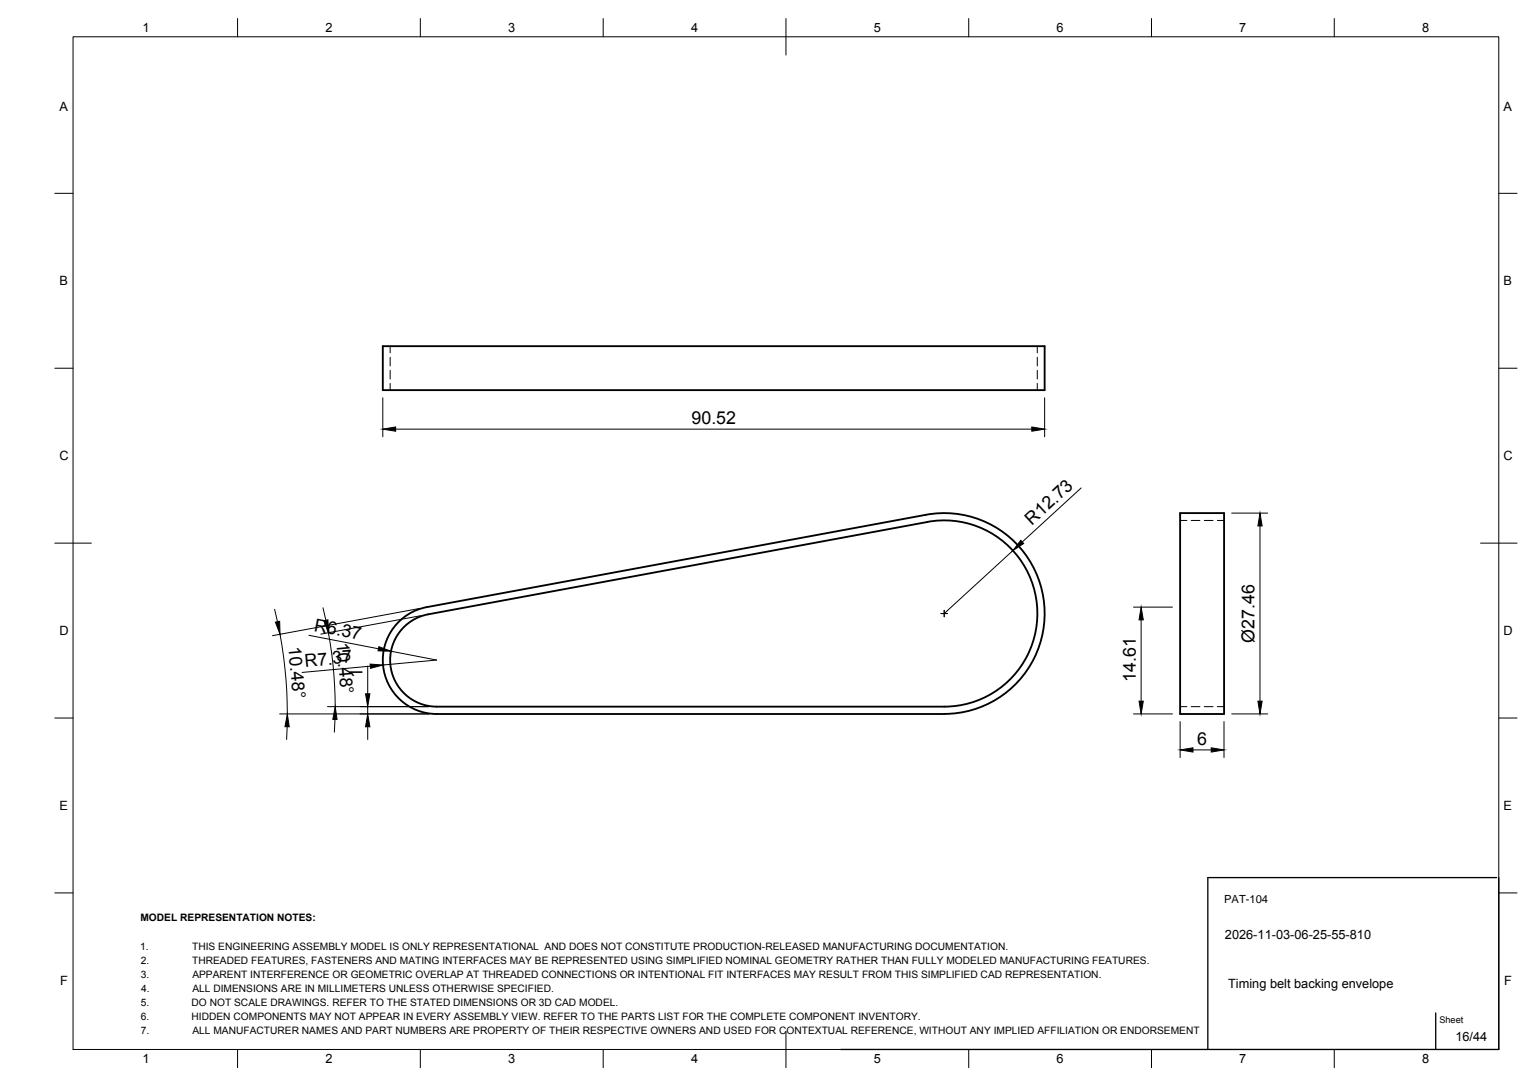
ISO-10303-21;
HEADER;
/* Generated by software containing ST-Developer
 * from STEP Tools, Inc. (www.steptools.com) 
 */

FILE_DESCRIPTION(
/* description */ ('Timing belt drive module 2 mm Pitch Timing 20T-40T'),

/* implementation_level */ '2;1');

FILE_NAME(
/* name */ 'Timing belt backing envelope.step',
/* time_stamp */ '2026-10-28T03:25:12-07:00',
/* author */ (''),
/* organization */ (''),
/* preprocessor_version */ 'ST-DEVELOPER v20.2',
/* originating_system */ 'Autodesk Translation Framework v15.17.0.0',
/* authorisation */ '');

FILE_SCHEMA (('AUTOMOTIVE_DESIGN { 1 0 10303 214 3 1 1 }'));
ENDSEC;

DATA;
#10=MECHANICAL_DESIGN_GEOMETRIC_PRESENTATION_REPRESENTATION('',(#539),#17830);
#453=SHAPE_REPRESENTATION_RELATIONSHIP('SRR','None',#18023,#496);
#496=ADVANCED_BREP_SHAPE_REPRESENTATION('',(#597),#17798);
#539=STYLED_ITEM('',(#18324),#597);
#597=MANIFOLD_SOLID_BREP('Body1',#8996);
#707=FACE_BOUND('',#1712,.T.);
#708=FACE_BOUND('',#1720,.T.);
#847=PLANE('',#9858);
#848=PLANE('',#9859);
#849=PLANE('',#9860);
#850=PLANE('',#9871);
#851=PLANE('',#9872);
#852=PLANE('',#9875);
#1118=FACE_OUTER_BOUND('',#1709,.T.);
#1119=FACE_OUTER_BOUND('',#1710,.T.);
#1120=FACE_OUTER_BOUND('',#1711,.T.);
#1121=FACE_OUTER_BOUND('',#1713,.T.);
#1122=FACE_OUTER_BOUND('',#1714,.T.);
#1123=FACE_OUTER_BOUND('',#1715,.T.);
#1124=FACE_OUTER_BOUND('',#1716,.T.);
#1125=FACE_OUTER_BOUND('',#1717,.T.);
#1126=FACE_OUTER_BOUND('',#1718,.T.);
#1127=FACE_OUTER_BOUND('',#1719,.T.);
#1709=EDGE_LOOP('',(#6493,#6494,#6495,#6496));
#1710=EDGE_LOOP('',(#6497,#6498,#6499,#6500));
#1711=EDGE_LOOP('',(#6501,#6502,#6503,#6504));
#1712=EDGE_LOOP('',(#6505,#6506,#6507,#6508));
#1713=EDGE_LOOP('',(#6509,#6510,#6511,#6512));
#1714=EDGE_LOOP('',(#6513,#6514,#6515,#6516));
#1715=EDGE_LOOP('',(#6517,#6518,#6519,#6520));
#1716=EDGE_LOOP('',(#6521,#6522,#6523,#6524));
#1717=EDGE_LOOP('',(#6525,#6526,#6527,#6528));
#1718=EDGE_LOOP('',(#6529,#6530,#6531,#6532));
#1719=EDGE_LOOP('',(#6533,#6534,#6535,#6536));
#1720=EDGE_LOOP('',(#6537,#6538,#6539,#6540));
#2308=CIRCLE('',#9861,0.736619772367581);
#2309=CIRCLE('',#9862,1.37323954473516);
#2310=CIRCLE('',#9863,0.636619772367581);
#2311=CIRCLE('',#9864,1.27323954473516);
#2312=CIRCLE('',#9866,0.636619772367581);
#2313=CIRCLE('',#9868,1.27323954473516);
#2314=CIRCLE('',#9870,1.37323954473516);
#2315=CIRCLE('',#9874,0.736619772367581);
#2982=LINE('',#14650,#3460);
#2983=LINE('',#14652,#3461);
#2984=LINE('',#14654,#3462);
#2985=LINE('',#14655,#3463);
#2986=LINE('',#14659,#3464);
#2987=LINE('',#14661,#3465);
#2988=LINE('',#14663,#3466);
#2989=LINE('',#14664,#3467);
#2990=LINE('',#14668,#3468);
#2991=LINE('',#14672,#3469);
#2992=LINE('',#14682,#3470);
#2993=LINE('',#14685,#3471);
#2994=LINE('',#14688,#3472);
#2995=LINE('',#14689,#3473);
#2996=LINE('',#14692,#3474);
#2997=LINE('',#14693,#3475);
#3460=VECTOR('',#11687,1.);
#3461=VECTOR('',#11688,1.);
#3462=VECTOR('',#11689,1.);
#3463=VECTOR('',#11690,1.);
#3464=VECTOR('',#11693,1.);
#3465=VECTOR('',#11694,1.);
#3466=VECTOR('',#11695,1.);
#3467=VECTOR('',#11696,1.);
#3468=VECTOR('',#11699,1.);
#3469=VECTOR('',#11702,1.);
#3470=VECTOR('',#11719,1.);
#3471=VECTOR('',#11722,1.);
#3472=VECTOR('',#11725,1.);
#3473=VECTOR('',#11726,1.);
#3474=VECTOR('',#11729,1.);
#3475=VECTOR('',#11730,1.);
#3986=VERTEX_POINT('',#14648);
#3987=VERTEX_POINT('',#14649);
#3988=VERTEX_POINT('',#14651);
#3989=VERTEX_POINT('',#14653);
#3990=VERTEX_POINT('',#14657);
#3991=VERTEX_POINT('',#14658);
#3992=VERTEX_POINT('',#14660);
#3993=VERTEX_POINT('',#14662);
#3994=VERTEX_POINT('',#14666);
#3995=VERTEX_POINT('',#14667);
#3996=VERTEX_POINT('',#14669);
#3997=VERTEX_POINT('',#14671);
#3998=VERTEX_POINT('',#14681);
#3999=VERTEX_POINT('',#14683);
#4000=VERTEX_POINT('',#14687);
#4001=VERTEX_POINT('',#14691);
#4929=EDGE_CURVE('',#3986,#3987,#2982,.T.);
#4930=EDGE_CURVE('',#3988,#3986,#2983,.T.);
#4931=EDGE_CURVE('',#3989,#3988,#2984,.T.);
#4932=EDGE_CURVE('',#3989,#3987,#2985,.T.);
#4933=EDGE_CURVE('',#3990,#3991,#2986,.T.);
#4934=EDGE_CURVE('',#3992,#3990,#2987,.T.);
#4935=EDGE_CURVE('',#3993,#3992,#2988,.T.);
#4936=EDGE_CURVE('',#3991,#3993,#2989,.T.);
#4937=EDGE_CURVE('',#3994,#3995,#2990,.T.);
#4938=EDGE_CURVE('',#3996,#3994,#2308,.T.);
#4939=EDGE_CURVE('',#3997,#3996,#2991,.T.);
#4940=EDGE_CURVE('',#3995,#3997,#2309,.T.);
#4941=EDGE_CURVE('',#3987,#3990,#2310,.T.);
#4942=EDGE_CURVE('',#3991,#3986,#2311,.T.);
#4943=EDGE_CURVE('',#3992,#3989,#2312,.T.);
#4944=EDGE_CURVE('',#3988,#3993,#2313,.T.);
#4945=EDGE_CURVE('',#3997,#3998,#2992,.T.);
#4946=EDGE_CURVE('',#3999,#3998,#2314,.T.);
#4947=EDGE_CURVE('',#3995,#3999,#2993,.T.);
#4948=EDGE_CURVE('',#3996,#4000,#2994,.T.);
#4949=EDGE_CURVE('',#3998,#4000,#2995,.T.);
#4950=EDGE_CURVE('',#4001,#3999,#2996,.T.);
#4951=EDGE_CURVE('',#3994,#4001,#2997,.T.);
#4952=EDGE_CURVE('',#4000,#4001,#2315,.T.);
#6493=ORIENTED_EDGE('',*,*,#4929,.F.);
#6494=ORIENTED_EDGE('',*,*,#4930,.F.);
#6495=ORIENTED_EDGE('',*,*,#4931,.F.);
#6496=ORIENTED_EDGE('',*,*,#4932,.T.);
#6497=ORIENTED_EDGE('',*,*,#4933,.F.);
#6498=ORIENTED_EDGE('',*,*,#4934,.F.);
#6499=ORIENTED_EDGE('',*,*,#4935,.F.);
#6500=ORIENTED_EDGE('',*,*,#4936,.F.);
#6501=ORIENTED_EDGE('',*,*,#4937,.F.);
#6502=ORIENTED_EDGE('',*,*,#4938,.F.);
#6503=ORIENTED_EDGE('',*,*,#4939,.F.);
#6504=ORIENTED_EDGE('',*,*,#4940,.F.);
#6505=ORIENTED_EDGE('',*,*,#4929,.T.);
#6506=ORIENTED_EDGE('',*,*,#4941,.T.);
#6507=ORIENTED_EDGE('',*,*,#4933,.T.);
#6508=ORIENTED_EDGE('',*,*,#4942,.T.);
#6509=ORIENTED_EDGE('',*,*,#4932,.F.);
#6510=ORIENTED_EDGE('',*,*,#4943,.F.);
#6511=ORIENTED_EDGE('',*,*,#4934,.T.);
#6512=ORIENTED_EDGE('',*,*,#4941,.F.);
#6513=ORIENTED_EDGE('',*,*,#4930,.T.);
#6514=ORIENTED_EDGE('',*,*,#4942,.F.);
#6515=ORIENTED_EDGE('',*,*,#4936,.T.);
#6516=ORIENTED_EDGE('',*,*,#4944,.F.);
#6517=ORIENTED_EDGE('',*,*,#4945,.T.);
#6518=ORIENTED_EDGE('',*,*,#4946,.F.);
#6519=ORIENTED_EDGE('',*,*,#4947,.F.);
#6520=ORIENTED_EDGE('',*,*,#4940,.T.);
#6521=ORIENTED_EDGE('',*,*,#4939,.T.);
#6522=ORIENTED_EDGE('',*,*,#4948,.T.);
#6523=ORIENTED_EDGE('',*,*,#4949,.F.);
#6524=ORIENTED_EDGE('',*,*,#4945,.F.);
#6525=ORIENTED_EDGE('',*,*,#4937,.T.);
#6526=ORIENTED_EDGE('',*,*,#4947,.T.);
#6527=ORIENTED_EDGE('',*,*,#4950,.F.);
#6528=ORIENTED_EDGE('',*,*,#4951,.F.);
#6529=ORIENTED_EDGE('',*,*,#4948,.F.);
#6530=ORIENTED_EDGE('',*,*,#4938,.T.);
#6531=ORIENTED_EDGE('',*,*,#4951,.T.);
#6532=ORIENTED_EDGE('',*,*,#4952,.F.);
#6533=ORIENTED_EDGE('',*,*,#4949,.T.);
#6534=ORIENTED_EDGE('',*,*,#4952,.T.);
#6535=ORIENTED_EDGE('',*,*,#4950,.T.);
#6536=ORIENTED_EDGE('',*,*,#4946,.T.);
#6537=ORIENTED_EDGE('',*,*,#4931,.T.);
#6538=ORIENTED_EDGE('',*,*,#4944,.T.);
#6539=ORIENTED_EDGE('',*,*,#4935,.T.);
#6540=ORIENTED_EDGE('',*,*,#4943,.T.);
#8263=CYLINDRICAL_SURFACE('',#9865,0.636619772367581);
#8264=CYLINDRICAL_SURFACE('',#9867,1.27323954473516);
#8265=CYLINDRICAL_SURFACE('',#9869,1.37323954473516);
#8266=CYLINDRICAL_SURFACE('',#9873,0.736619772367581);
#8616=ADVANCED_FACE('',(#1118),#847,.F.);
#8617=ADVANCED_FACE('',(#1119),#848,.F.);
#8618=ADVANCED_FACE('',(#1120,#707),#849,.F.);
#8619=ADVANCED_FACE('',(#1121),#8263,.F.);
#8620=ADVANCED_FACE('',(#1122),#8264,.F.);
#8621=ADVANCED_FACE('',(#1123),#8265,.T.);
#8622=ADVANCED_FACE('',(#1124),#850,.T.);
#8623=ADVANCED_FACE('',(#1125),#851,.T.);
#8624=ADVANCED_FACE('',(#1126),#8266,.T.);
#8625=ADVANCED_FACE('',(#1127,#708),#852,.T.);
#8996=CLOSED_SHELL('',(#8616,#8617,#8618,#8619,#8620,#8621,#8622,#8623,
#8624,#8625));
#9857=AXIS2_PLACEMENT_3D('',#14646,#11683,#11684);
#9858=AXIS2_PLACEMENT_3D('',#14647,#11685,#11686);
#9859=AXIS2_PLACEMENT_3D('',#14656,#11691,#11692);
#9860=AXIS2_PLACEMENT_3D('',#14665,#11697,#11698);
#9861=AXIS2_PLACEMENT_3D('',#14670,#11700,#11701);
#9862=AXIS2_PLACEMENT_3D('',#14673,#11703,#11704);
#9863=AXIS2_PLACEMENT_3D('',#14674,#11705,#11706);
#9864=AXIS2_PLACEMENT_3D('',#14675,#11707,#11708);
#9865=AXIS2_PLACEMENT_3D('',#14676,#11709,#11710);
#9866=AXIS2_PLACEMENT_3D('',#14677,#11711,#11712);
#9867=AXIS2_PLACEMENT_3D('',#14678,#11713,#11714);
#9868=AXIS2_PLACEMENT_3D('',#14679,#11715,#11716);
#9869=AXIS2_PLACEMENT_3D('',#14680,#11717,#11718);
#9870=AXIS2_PLACEMENT_3D('',#14684,#11720,#11721);
#9871=AXIS2_PLACEMENT_3D('',#14686,#11723,#11724);
#9872=AXIS2_PLACEMENT_3D('',#14690,#11727,#11728);
#9873=AXIS2_PLACEMENT_3D('',#14694,#11731,#11732);
#9874=AXIS2_PLACEMENT_3D('',#14695,#11733,#11734);
#9875=AXIS2_PLACEMENT_3D('',#14696,#11735,#11736);
#11683=DIRECTION('axis',(0.,0.,1.));
#11684=DIRECTION('refdir',(1.,0.,0.));
#11685=DIRECTION('center_axis',(-0.0913252028230577,0.,-0.99582112215464));
#11686=DIRECTION('ref_axis',(-0.99582112215464,0.,0.0913252028230577));
#11687=DIRECTION('',(-0.99582112215464,0.,0.0913252028230577));
#11688=DIRECTION('',(0.,-1.,0.));
#11689=DIRECTION('',(0.99582112215464,0.,-0.0913252028230577));
#11690=DIRECTION('',(0.,-1.,0.));
#11691=DIRECTION('center_axis',(-0.0913252028230577,0.,0.99582112215464));
#11692=DIRECTION('ref_axis',(0.99582112215464,0.,0.0913252028230577));
#11693=DIRECTION('',(0.99582112215464,0.,0.0913252028230577));
#11694=DIRECTION('',(0.,-1.,0.));
#11695=DIRECTION('',(-0.99582112215464,0.,-0.0913252028230577));
#11696=DIRECTION('',(0.,1.,0.));
#11697=DIRECTION('center_axis',(0.,1.,0.));
#11698=DIRECTION('ref_axis',(1.,0.,0.));
#11699=DIRECTION('',(0.99582112215464,0.,0.091325202823058));
#11700=DIRECTION('center_axis',(0.,1.,0.));
#11701=DIRECTION('ref_axis',(1.,0.,0.));
#11702=DIRECTION('',(-0.99582112215464,0.,0.0913252028230577));
#11703=DIRECTION('center_axis',(0.,1.,0.));
#11704=DIRECTION('ref_axis',(1.,0.,0.));
#11705=DIRECTION('center_axis',(0.,1.,0.));
#11706=DIRECTION('ref_axis',(1.,0.,0.));
#11707=DIRECTION('center_axis',(0.,1.,0.));
#11708=DIRECTION('ref_axis',(1.,0.,0.));
#11709=DIRECTION('center_axis',(0.,1.,0.));
#11710=DIRECTION('ref_axis',(-1.,0.,-1.22464679914735E-16));
#11711=DIRECTION('center_axis',(0.,-1.,0.));
#11712=DIRECTION('ref_axis',(1.,0.,0.));
#11713=DIRECTION('center_axis',(0.,1.,0.));
#11714=DIRECTION('ref_axis',(1.,0.,0.));
#11715=DIRECTION('center_axis',(0.,-1.,0.));
#11716=DIRECTION('ref_axis',(1.,0.,0.));
#11717=DIRECTION('center_axis',(0.,1.,0.));
#11718=DIRECTION('ref_axis',(1.,0.,0.));
#11719=DIRECTION('',(0.,1.,0.));
#11720=DIRECTION('center_axis',(0.,1.,0.));
#11721=DIRECTION('ref_axis',(1.,0.,0.));
#11722=DIRECTION('',(0.,1.,0.));
#11723=DIRECTION('center_axis',(-0.0913252028230577,0.,-0.99582112215464));
#11724=DIRECTION('ref_axis',(-0.99582112215464,0.,0.0913252028230577));
#11725=DIRECTION('',(0.,1.,0.));
#11726=DIRECTION('',(-0.99582112215464,0.,0.0913252028230577));
#11727=DIRECTION('center_axis',(-0.091325202823058,0.,0.99582112215464));
#11728=DIRECTION('ref_axis',(0.99582112215464,0.,0.091325202823058));
#11729=DIRECTION('',(0.99582112215464,0.,0.091325202823058));
#11730=DIRECTION('',(0.,1.,0.));
#11731=DIRECTION('center_axis',(0.,1.,0.));
#11732=DIRECTION('ref_axis',(-1.,0.,-1.22464679914735E-16));
#11733=DIRECTION('center_axis',(0.,1.,0.));
#11734=DIRECTION('ref_axis',(1.,0.,0.));
#11735=DIRECTION('center_axis',(0.,1.,0.));
#11736=DIRECTION('ref_axis',(1.,0.,0.));
#14646=CARTESIAN_POINT('',(0.,0.,0.));
#14647=CARTESIAN_POINT('Origin',(6.85463117051588,-3.5,5.73208116779017));
#14648=CARTESIAN_POINT('',(6.85463117051588,-3.425,5.73208116779017));
#14649=CARTESIAN_POINT('',(-0.0581394298326381,-3.425,6.36604058389508));
#14650=CARTESIAN_POINT('',(3.39824587034162,-3.425,6.04906087584262));
#14651=CARTESIAN_POINT('',(6.85463117051588,-2.825,5.73208116779017));
#14652=CARTESIAN_POINT('',(6.85463117051588,-3.5,5.73208116779017));
#14653=CARTESIAN_POINT('',(-0.0581394298326381,-2.825,6.36604058389508));
#14654=CARTESIAN_POINT('',(3.39824587034162,-2.825,6.04906087584262));
#14655=CARTESIAN_POINT('',(-0.0581394298326381,-3.5,6.36604058389508));
#14656=CARTESIAN_POINT('Origin',(-0.0581394298326382,-3.5,7.63395941610492));
#14657=CARTESIAN_POINT('',(-0.0581394298326382,-3.425,7.63395941610492));
#14658=CARTESIAN_POINT('',(6.85463117051588,-3.425,8.26791883220983));
#14659=CARTESIAN_POINT('',(-0.0581394298326382,-3.425,7.63395941610492));
#14660=CARTESIAN_POINT('',(-0.0581394298326382,-2.825,7.63395941610492));
#14661=CARTESIAN_POINT('',(-0.0581394298326382,-3.5,7.63395941610492));
#14662=CARTESIAN_POINT('',(6.85463117051588,-2.825,8.26791883220983));
#14663=CARTESIAN_POINT('',(-0.0581394298326382,-2.825,7.63395941610492));
#14664=CARTESIAN_POINT('',(6.85463117051588,-3.5,8.26791883220983));
#14665=CARTESIAN_POINT('Origin',(0.,-3.425,7.));
#14666=CARTESIAN_POINT('',(-0.067271950114944,-3.425,7.73354152832038));
#14667=CARTESIAN_POINT('',(6.84549865023357,-3.425,8.3675009444253));
#14668=CARTESIAN_POINT('',(-0.067271950114944,-3.425,7.73354152832038));
#14669=CARTESIAN_POINT('',(-0.067271950114944,-3.425,6.26645847167962));
#14670=CARTESIAN_POINT('Origin',(0.,-3.425,7.));
#14671=CARTESIAN_POINT('',(6.84549865023357,-3.425,5.6324990555747));
#14672=CARTESIAN_POINT('',(6.84549865023357,-3.425,5.6324990555747));
#14673=CARTESIAN_POINT('Origin',(6.97091003018116,-3.425,7.));
#14674=CARTESIAN_POINT('Origin',(0.,-3.425,7.));
#14675=CARTESIAN_POINT('Origin',(6.97091003018116,-3.425,7.));
#14676=CARTESIAN_POINT('Origin',(0.,-3.5,7.));
#14677=CARTESIAN_POINT('Origin',(0.,-2.825,7.));
#14678=CARTESIAN_POINT('Origin',(6.97091003018116,-3.5,7.));
#14679=CARTESIAN_POINT('Origin',(6.97091003018116,-2.825,7.));
#14680=CARTESIAN_POINT('Origin',(6.97091003018116,-3.425,7.));
#14681=CARTESIAN_POINT('',(6.84549865023357,-2.825,5.6324990555747));
#14682=CARTESIAN_POINT('',(6.84549865023357,-3.425,5.6324990555747));
#14683=CARTESIAN_POINT('',(6.84549865023357,-2.825,8.3675009444253));
#14684=CARTESIAN_POINT('Origin',(6.97091003018116,-2.825,7.));
#14685=CARTESIAN_POINT('',(6.84549865023357,-3.425,8.3675009444253));
#14686=CARTESIAN_POINT('Origin',(6.84549865023357,-3.425,5.6324990555747));
#14687=CARTESIAN_POINT('',(-0.067271950114944,-2.825,6.26645847167962));
#14688=CARTESIAN_POINT('',(-0.0672719501149439,-3.425,6.26645847167962));
#14689=CARTESIAN_POINT('',(6.84549865023357,-2.825,5.6324990555747));
#14690=CARTESIAN_POINT('Origin',(-0.067271950114944,-3.425,7.73354152832038));
#14691=CARTESIAN_POINT('',(-0.067271950114944,-2.825,7.73354152832038));
#14692=CARTESIAN_POINT('',(-0.067271950114944,-2.825,7.73354152832038));
#14693=CARTESIAN_POINT('',(-0.0672719501149441,-3.425,7.73354152832038));
#14694=CARTESIAN_POINT('Origin',(0.,-3.425,7.));
#14695=CARTESIAN_POINT('Origin',(0.,-2.825,7.));
#14696=CARTESIAN_POINT('Origin',(0.,-2.825,7.));
#17748=UNCERTAINTY_MEASURE_WITH_UNIT(LENGTH_MEASURE(0.001),#17831,
'DISTANCE_ACCURACY_VALUE',
'Maximum model space distance between geometric entities at asserted c
onnectivities');
#17780=UNCERTAINTY_MEASURE_WITH_UNIT(LENGTH_MEASURE(0.001),#17831,
'DISTANCE_ACCURACY_VALUE',
'Maximum model space distance between geometric entities at asserted c
onnectivities');
#17798=(
GEOMETRIC_REPRESENTATION_CONTEXT(3)
GLOBAL_UNCERTAINTY_ASSIGNED_CONTEXT((#17748))
GLOBAL_UNIT_ASSIGNED_CONTEXT((#17831,#17833,#17834))
REPRESENTATION_CONTEXT('','3D')
);
#17830=(
GEOMETRIC_REPRESENTATION_CONTEXT(3)
GLOBAL_UNCERTAINTY_ASSIGNED_CONTEXT((#17780))
GLOBAL_UNIT_ASSIGNED_CONTEXT((#17831,#17833,#17834))
REPRESENTATION_CONTEXT('','3D')
);
#17831=(
LENGTH_UNIT()
NAMED_UNIT(*)
SI_UNIT(.CENTI.,.METRE.)
);
#17833=(
NAMED_UNIT(*)
PLANE_ANGLE_UNIT()
SI_UNIT($,.RADIAN.)
);
#17834=(
NAMED_UNIT(*)
SI_UNIT($,.STERADIAN.)
SOLID_ANGLE_UNIT()
);
#17852=SHAPE_DEFINITION_REPRESENTATION(#17901,#18023);
#17901=PRODUCT_DEFINITION_SHAPE('',$,#18073);
#18023=SHAPE_REPRESENTATION('',(#9857),#17798);
#18055=PRODUCT_DEFINITION_CONTEXT('part definition',#18204,'design');
#18073=PRODUCT_DEFINITION('Timing belt backing envelope',
'Timing belt backing envelope',#18122,#18055);
#18122=PRODUCT_DEFINITION_FORMATION('',$,#18223);
#18204=APPLICATION_CONTEXT(
'Core Data for Automotive Mechanical Design Process');
#18205=PRODUCT_CONTEXT('part definition',#18204,'mechanical');
#18223=PRODUCT('Timing belt backing envelope',
'Timing belt backing envelope','Timing belt backing envelope',(#18205));
#18318=COLOUR_RGB('Black',0.12,0.14,0.17);
#18319=FILL_AREA_STYLE_COLOUR('',#18318);
#18320=FILL_AREA_STYLE('',(#18319));
#18321=SURFACE_STYLE_FILL_AREA(#18320);
#18322=SURFACE_SIDE_STYLE('',(#18321));
#18323=SURFACE_STYLE_USAGE(.BOTH.,#18322);
#18324=PRESENTATION_STYLE_ASSIGNMENT((#18323));
ENDSEC;
END-ISO-10303-21;
